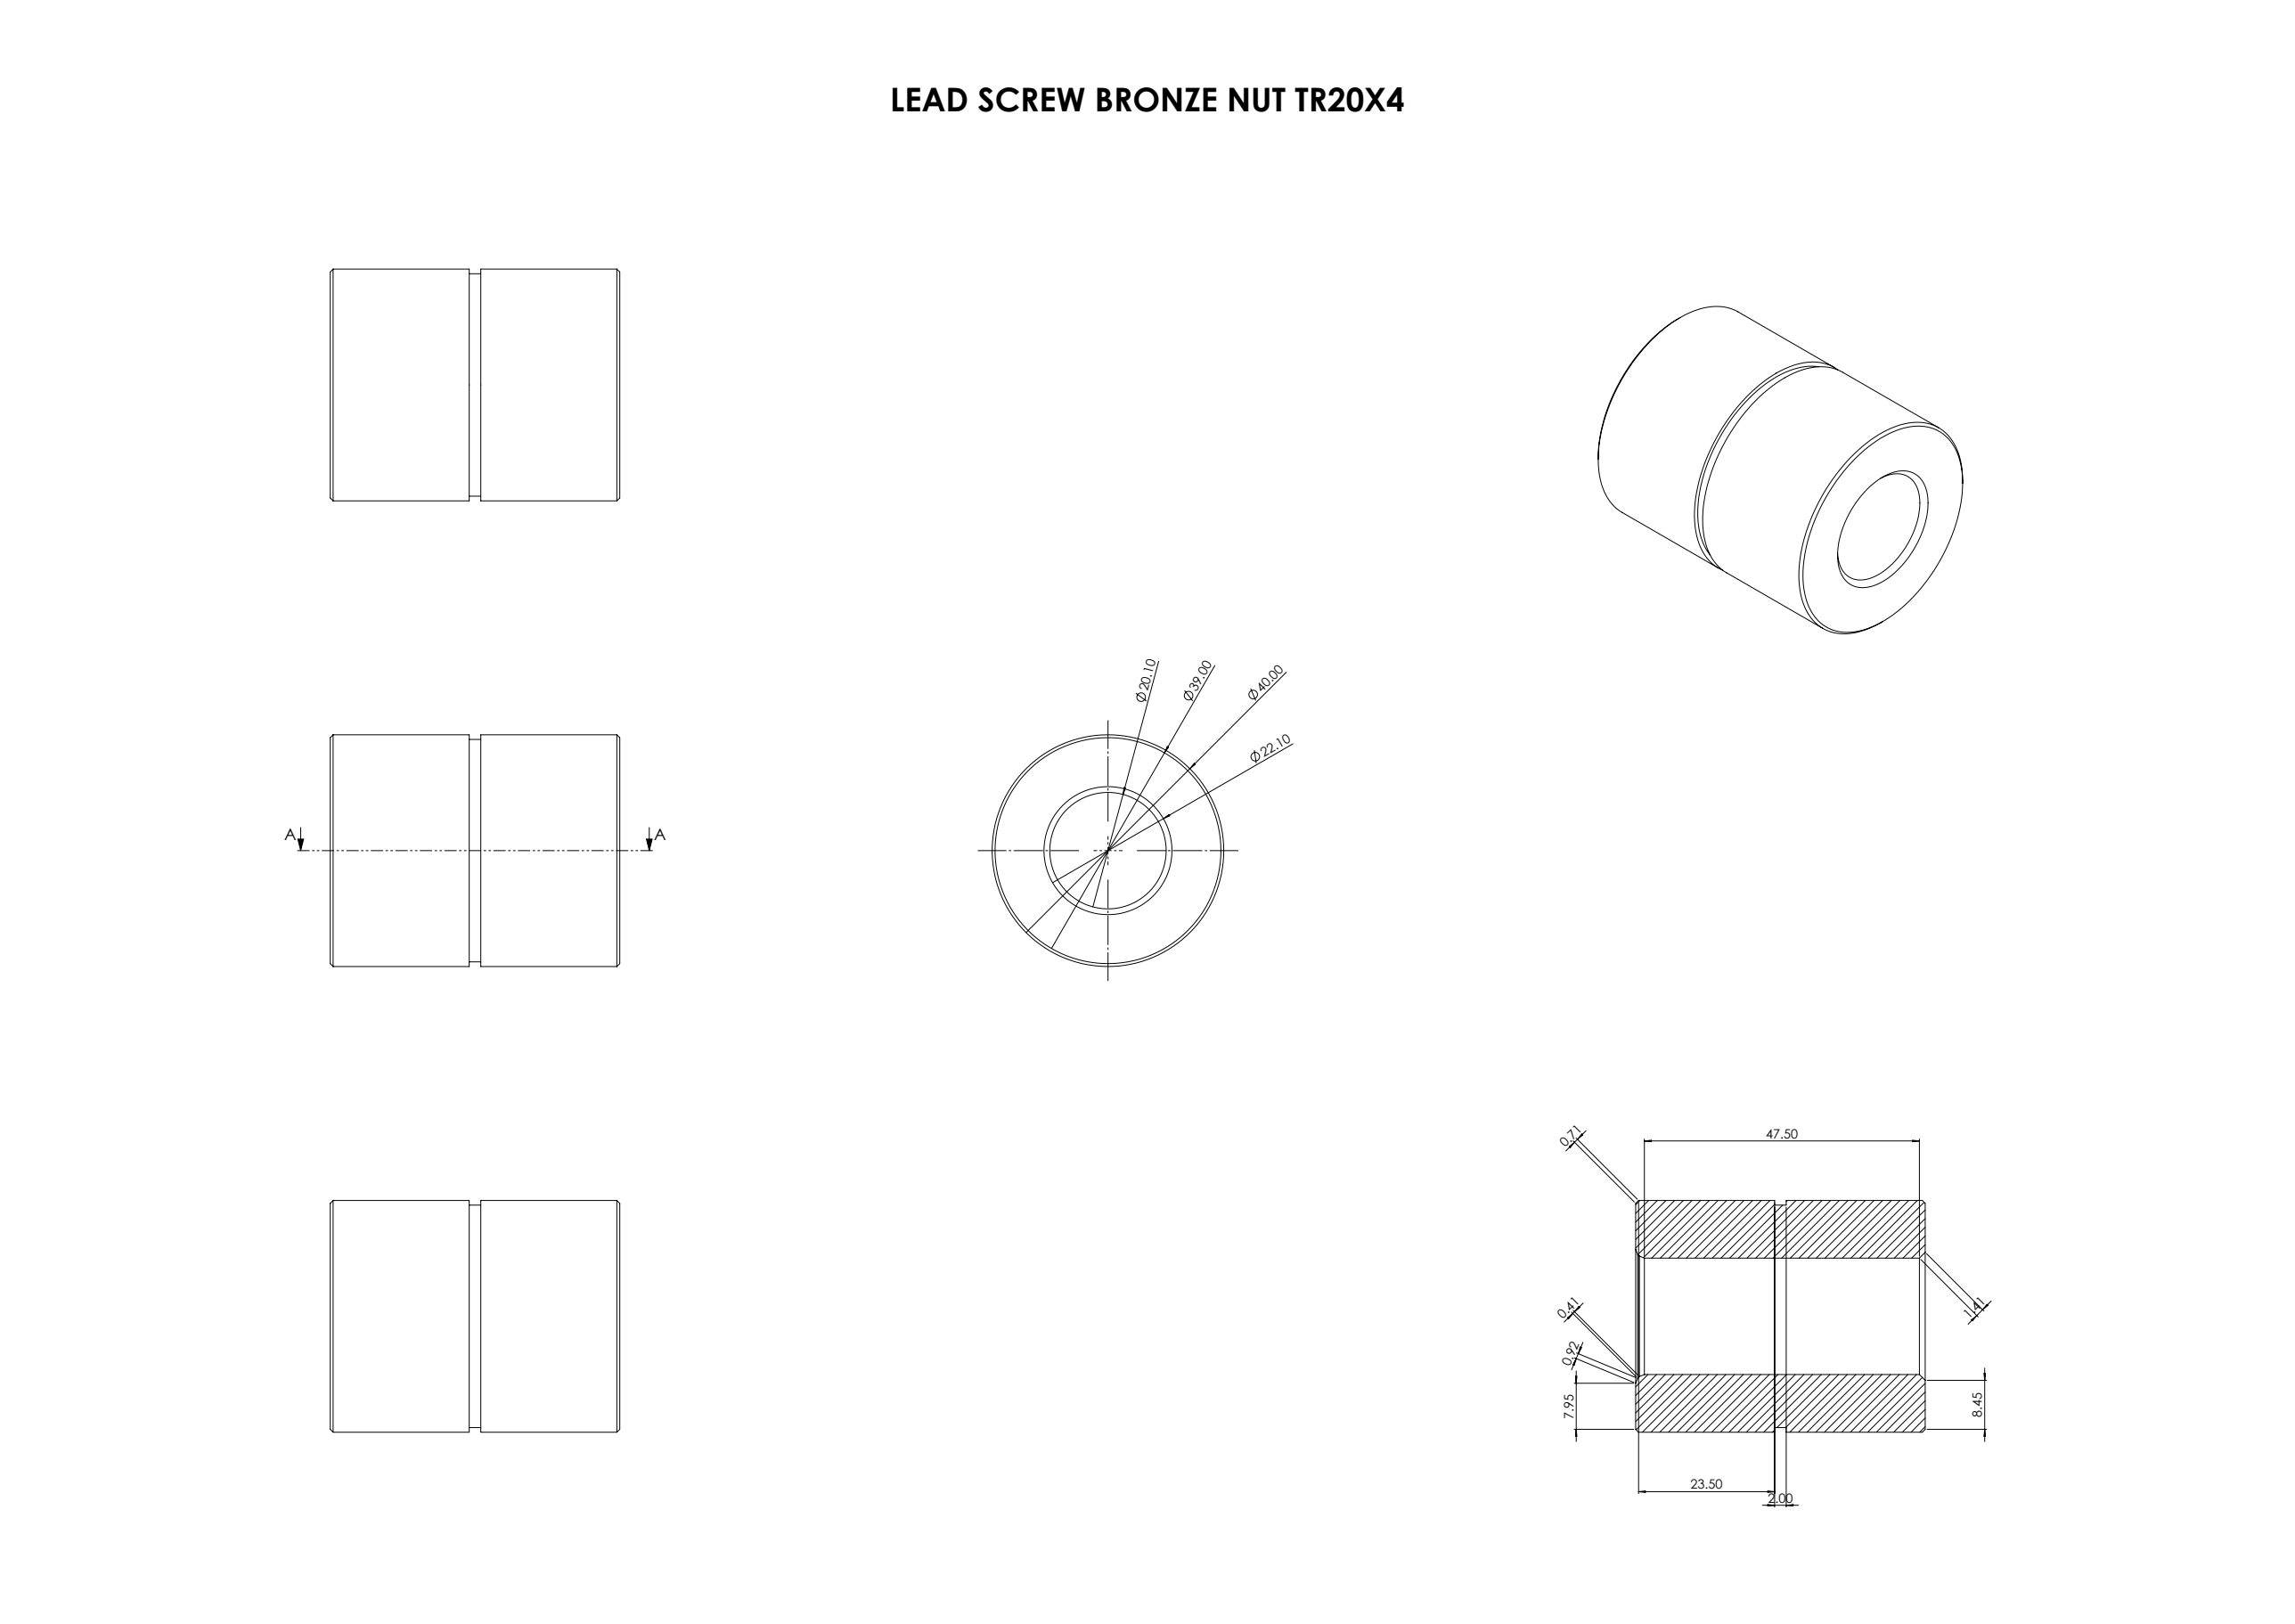
ISO-10303-21;
HEADER;
/* Generated by software containing ST-Developer
 * from STEP Tools, Inc. (www.steptools.com) 
 */

FILE_DESCRIPTION(
/* description */ (''),
/* implementation_level */ '2;1');

FILE_NAME(
/* name */ '06_Lead_Screw_Bronze_Nut_Tr20x4.step',
/* time_stamp */ '2026-10-26T03:50:32-07:00',
/* author */ (''),
/* organization */ (''),
/* preprocessor_version */ 'ST-DEVELOPER v20.2',
/* originating_system */ 'Autodesk Translation Framework v15.15.0.0',
/* authorisation */ '');

FILE_SCHEMA (('AUTOMOTIVE_DESIGN { 1 0 10303 214 3 1 1 }'));
ENDSEC;

DATA;
#10=MECHANICAL_DESIGN_GEOMETRIC_PRESENTATION_REPRESENTATION('',(#1044),#76660);
#1004=SHAPE_REPRESENTATION_RELATIONSHIP('SRR','None',#76741,#1024);
#1024=ADVANCED_BREP_SHAPE_REPRESENTATION('',(#1064),#76645);
#1044=STYLED_ITEM('',(#76913),#1064);
#1064=MANIFOLD_SOLID_BREP('Bronze nut',#26669);
#1251=CYLINDRICAL_SURFACE('',#27734,1.005);
#1252=CYLINDRICAL_SURFACE('',#27739,1.92);
#1253=CYLINDRICAL_SURFACE('',#27743,2.);
#1254=CYLINDRICAL_SURFACE('',#27746,2.);
#1610=FACE_BOUND('',#4683,.T.);
#1611=FACE_BOUND('',#4687,.T.);
#1612=FACE_BOUND('',#4690,.T.);
#1613=FACE_BOUND('',#4696,.T.);
#1925=PLANE('',#27729);
#1926=PLANE('',#27736);
#1927=PLANE('',#27741);
#1928=PLANE('',#27750);
#3071=FACE_OUTER_BOUND('',#4680,.T.);
#3072=FACE_OUTER_BOUND('',#4681,.T.);
#3073=FACE_OUTER_BOUND('',#4682,.T.);
#3074=FACE_OUTER_BOUND('',#4684,.T.);
#3075=FACE_OUTER_BOUND('',#4685,.T.);
#3076=FACE_OUTER_BOUND('',#4686,.T.);
#3077=FACE_OUTER_BOUND('',#4688,.T.);
#3078=FACE_OUTER_BOUND('',#4689,.T.);
#3079=FACE_OUTER_BOUND('',#4691,.T.);
#3080=FACE_OUTER_BOUND('',#4692,.T.);
#3081=FACE_OUTER_BOUND('',#4693,.T.);
#3082=FACE_OUTER_BOUND('',#4694,.T.);
#3083=FACE_OUTER_BOUND('',#4695,.T.);
#3084=FACE_OUTER_BOUND('',#4697,.T.);
#4680=EDGE_LOOP('',(#19859,#19860,#19861,#19862,#19863));
#4681=EDGE_LOOP('',(#19864,#19865,#19866,#19867,#19868,#19869));
#4682=EDGE_LOOP('',(#19870));
#4683=EDGE_LOOP('',(#19871));
#4684=EDGE_LOOP('',(#19872,#19873,#19874,#19875,#19876,#19877));
#4685=EDGE_LOOP('',(#19878,#19879,#19880,#19881,#19882));
#4686=EDGE_LOOP('',(#19883));
#4687=EDGE_LOOP('',(#19884));
#4688=EDGE_LOOP('',(#19885,#19886,#19887,#19888));
#4689=EDGE_LOOP('',(#19889));
#4690=EDGE_LOOP('',(#19890));
#4691=EDGE_LOOP('',(#19891,#19892,#19893,#19894));
#4692=EDGE_LOOP('',(#19895,#19896,#19897,#19898));
#4693=EDGE_LOOP('',(#19899,#19900,#19901,#19902));
#4694=EDGE_LOOP('',(#19903,#19904,#19905,#19906));
#4695=EDGE_LOOP('',(#19907));
#4696=EDGE_LOOP('',(#19908));
#4697=EDGE_LOOP('',(#19909,#19910,#19911,#19912));
#6006=CIRCLE('',#27723,1.155);
#6007=CIRCLE('',#27724,1.06964466094067);
#6008=CIRCLE('',#27725,1.06964466094067);
#6009=CIRCLE('',#27727,1.04035533905933);
#6010=CIRCLE('',#27728,1.04035533905933);
#6011=CIRCLE('',#27730,1.95);
#6012=CIRCLE('',#27732,1.005);
#6013=CIRCLE('',#27733,1.005);
#6014=CIRCLE('',#27735,1.005);
#6015=CIRCLE('',#27737,2.);
#6016=CIRCLE('',#27738,1.92);
#6017=CIRCLE('',#27740,1.92);
#6018=CIRCLE('',#27742,2.);
#6019=CIRCLE('',#27744,2.);
#6020=CIRCLE('',#27747,2.);
#6021=CIRCLE('',#27749,1.95);
#6022=CIRCLE('',#27751,1.105);
#7397=LINE('',#49634,#9553);
#7398=LINE('',#49643,#9554);
#7399=LINE('',#49649,#9555);
#7400=LINE('',#49656,#9556);
#7401=LINE('',#49665,#9557);
#7402=LINE('',#49671,#9558);
#7403=LINE('',#49674,#9559);
#7404=LINE('',#49678,#9560);
#7405=LINE('',#49682,#9561);
#7406=LINE('',#49687,#9562);
#9553=VECTOR('',#31788,1.11232233047034);
#9554=VECTOR('',#31799,1.055);
#9555=VECTOR('',#31806,1.02267766952966);
#9556=VECTOR('',#31815,1.005);
#9557=VECTOR('',#31826,1.92);
#9558=VECTOR('',#31833,2.);
#9559=VECTOR('',#31838,1.975);
#9560=VECTOR('',#31843,2.);
#9561=VECTOR('',#31848,1.975);
#9562=VECTOR('',#31855,1.055);
#11737=VERTEX_POINT('',#49631);
#11738=VERTEX_POINT('',#49633);
#11739=VERTEX_POINT('',#49635);
#11740=VERTEX_POINT('',#49639);
#11741=VERTEX_POINT('',#49640);
#11742=VERTEX_POINT('',#49645);
#11743=VERTEX_POINT('',#49648);
#11744=VERTEX_POINT('',#49650);
#11745=VERTEX_POINT('',#49654);
#11746=VERTEX_POINT('',#49658);
#11747=VERTEX_POINT('',#49660);
#11748=VERTEX_POINT('',#49663);
#11749=VERTEX_POINT('',#49667);
#11750=VERTEX_POINT('',#49670);
#11751=VERTEX_POINT('',#49676);
#11752=VERTEX_POINT('',#49680);
#11753=VERTEX_POINT('',#49684);
#14652=EDGE_CURVE('',#11737,#11737,#6006,.T.);
#14653=EDGE_CURVE('',#11737,#11738,#7397,.T.);
#14654=EDGE_CURVE('',#11738,#11739,#6007,.T.);
#14655=EDGE_CURVE('',#11739,#11738,#6008,.T.);
#14656=EDGE_CURVE('',#11740,#11741,#6009,.T.);
#14657=EDGE_CURVE('',#11741,#11740,#6010,.T.);
#14658=EDGE_CURVE('',#11741,#11739,#7398,.T.);
#14659=EDGE_CURVE('',#11742,#11742,#6011,.T.);
#14660=EDGE_CURVE('',#11740,#11743,#7399,.T.);
#14661=EDGE_CURVE('',#11743,#11744,#6012,.T.);
#14662=EDGE_CURVE('',#11744,#11743,#6013,.T.);
#14663=EDGE_CURVE('',#11745,#11745,#6014,.T.);
#14664=EDGE_CURVE('',#11745,#11744,#7400,.T.);
#14665=EDGE_CURVE('',#11746,#11746,#6015,.T.);
#14666=EDGE_CURVE('',#11747,#11747,#6016,.T.);
#14667=EDGE_CURVE('',#11748,#11748,#6017,.T.);
#14668=EDGE_CURVE('',#11748,#11747,#7401,.T.);
#14669=EDGE_CURVE('',#11749,#11749,#6018,.T.);
#14670=EDGE_CURVE('',#11749,#11750,#7402,.T.);
#14671=EDGE_CURVE('',#11750,#11750,#6019,.T.);
#14672=EDGE_CURVE('',#11750,#11742,#7403,.T.);
#14673=EDGE_CURVE('',#11751,#11751,#6020,.T.);
#14674=EDGE_CURVE('',#11751,#11746,#7404,.T.);
#14675=EDGE_CURVE('',#11752,#11752,#6021,.T.);
#14676=EDGE_CURVE('',#11752,#11751,#7405,.T.);
#14677=EDGE_CURVE('',#11753,#11753,#6022,.T.);
#14678=EDGE_CURVE('',#11753,#11745,#7406,.T.);
#19859=ORIENTED_EDGE('',*,*,#14652,.T.);
#19860=ORIENTED_EDGE('',*,*,#14653,.T.);
#19861=ORIENTED_EDGE('',*,*,#14654,.T.);
#19862=ORIENTED_EDGE('',*,*,#14655,.T.);
#19863=ORIENTED_EDGE('',*,*,#14653,.F.);
#19864=ORIENTED_EDGE('',*,*,#14656,.F.);
#19865=ORIENTED_EDGE('',*,*,#14657,.F.);
#19866=ORIENTED_EDGE('',*,*,#14658,.T.);
#19867=ORIENTED_EDGE('',*,*,#14654,.F.);
#19868=ORIENTED_EDGE('',*,*,#14655,.F.);
#19869=ORIENTED_EDGE('',*,*,#14658,.F.);
#19870=ORIENTED_EDGE('',*,*,#14659,.F.);
#19871=ORIENTED_EDGE('',*,*,#14652,.F.);
#19872=ORIENTED_EDGE('',*,*,#14656,.T.);
#19873=ORIENTED_EDGE('',*,*,#14657,.T.);
#19874=ORIENTED_EDGE('',*,*,#14660,.T.);
#19875=ORIENTED_EDGE('',*,*,#14661,.T.);
#19876=ORIENTED_EDGE('',*,*,#14662,.T.);
#19877=ORIENTED_EDGE('',*,*,#14660,.F.);
#19878=ORIENTED_EDGE('',*,*,#14663,.T.);
#19879=ORIENTED_EDGE('',*,*,#14664,.T.);
#19880=ORIENTED_EDGE('',*,*,#14661,.F.);
#19881=ORIENTED_EDGE('',*,*,#14662,.F.);
#19882=ORIENTED_EDGE('',*,*,#14664,.F.);
#19883=ORIENTED_EDGE('',*,*,#14665,.F.);
#19884=ORIENTED_EDGE('',*,*,#14666,.T.);
#19885=ORIENTED_EDGE('',*,*,#14667,.T.);
#19886=ORIENTED_EDGE('',*,*,#14668,.T.);
#19887=ORIENTED_EDGE('',*,*,#14666,.F.);
#19888=ORIENTED_EDGE('',*,*,#14668,.F.);
#19889=ORIENTED_EDGE('',*,*,#14669,.F.);
#19890=ORIENTED_EDGE('',*,*,#14667,.F.);
#19891=ORIENTED_EDGE('',*,*,#14669,.T.);
#19892=ORIENTED_EDGE('',*,*,#14670,.T.);
#19893=ORIENTED_EDGE('',*,*,#14671,.T.);
#19894=ORIENTED_EDGE('',*,*,#14670,.F.);
#19895=ORIENTED_EDGE('',*,*,#14671,.F.);
#19896=ORIENTED_EDGE('',*,*,#14672,.T.);
#19897=ORIENTED_EDGE('',*,*,#14659,.T.);
#19898=ORIENTED_EDGE('',*,*,#14672,.F.);
#19899=ORIENTED_EDGE('',*,*,#14673,.F.);
#19900=ORIENTED_EDGE('',*,*,#14674,.T.);
#19901=ORIENTED_EDGE('',*,*,#14665,.T.);
#19902=ORIENTED_EDGE('',*,*,#14674,.F.);
#19903=ORIENTED_EDGE('',*,*,#14675,.F.);
#19904=ORIENTED_EDGE('',*,*,#14676,.T.);
#19905=ORIENTED_EDGE('',*,*,#14673,.T.);
#19906=ORIENTED_EDGE('',*,*,#14676,.F.);
#19907=ORIENTED_EDGE('',*,*,#14675,.T.);
#19908=ORIENTED_EDGE('',*,*,#14677,.F.);
#19909=ORIENTED_EDGE('',*,*,#14677,.T.);
#19910=ORIENTED_EDGE('',*,*,#14678,.T.);
#19911=ORIENTED_EDGE('',*,*,#14663,.F.);
#19912=ORIENTED_EDGE('',*,*,#14678,.F.);
#25027=CONICAL_SURFACE('',#27722,1.11232233047034,1.17809724509617);
#25028=CONICAL_SURFACE('',#27726,1.055,0.78539816339745);
#25029=CONICAL_SURFACE('',#27731,1.02267766952966,0.39269908169873);
#25030=CONICAL_SURFACE('',#27745,1.975,0.785398163397442);
#25031=CONICAL_SURFACE('',#27748,1.975,0.785398163397442);
#25032=CONICAL_SURFACE('',#27752,1.055,0.78539816339745);
#25659=ADVANCED_FACE('',(#3071),#25027,.F.);
#25660=ADVANCED_FACE('',(#3072),#25028,.F.);
#25661=ADVANCED_FACE('',(#3073,#1610),#1925,.T.);
#25662=ADVANCED_FACE('',(#3074),#25029,.F.);
#25663=ADVANCED_FACE('',(#3075),#1251,.F.);
#25664=ADVANCED_FACE('',(#3076,#1611),#1926,.F.);
#25665=ADVANCED_FACE('',(#3077),#1252,.T.);
#25666=ADVANCED_FACE('',(#3078,#1612),#1927,.F.);
#25667=ADVANCED_FACE('',(#3079),#1253,.T.);
#25668=ADVANCED_FACE('',(#3080),#25030,.T.);
#25669=ADVANCED_FACE('',(#3081),#1254,.T.);
#25670=ADVANCED_FACE('',(#3082),#25031,.T.);
#25671=ADVANCED_FACE('',(#3083,#1613),#1928,.T.);
#25672=ADVANCED_FACE('',(#3084),#25032,.F.);
#26669=CLOSED_SHELL('',(#25659,#25660,#25661,#25662,#25663,#25664,#25665,
#25666,#25667,#25668,#25669,#25670,#25671,#25672));
#27721=AXIS2_PLACEMENT_3D('',#49629,#31782,#31783);
#27722=AXIS2_PLACEMENT_3D('',#49630,#31784,#31785);
#27723=AXIS2_PLACEMENT_3D('',#49632,#31786,#31787);
#27724=AXIS2_PLACEMENT_3D('',#49636,#31789,#31790);
#27725=AXIS2_PLACEMENT_3D('',#49637,#31791,#31792);
#27726=AXIS2_PLACEMENT_3D('',#49638,#31793,#31794);
#27727=AXIS2_PLACEMENT_3D('',#49641,#31795,#31796);
#27728=AXIS2_PLACEMENT_3D('',#49642,#31797,#31798);
#27729=AXIS2_PLACEMENT_3D('',#49644,#31800,#31801);
#27730=AXIS2_PLACEMENT_3D('',#49646,#31802,#31803);
#27731=AXIS2_PLACEMENT_3D('',#49647,#31804,#31805);
#27732=AXIS2_PLACEMENT_3D('',#49651,#31807,#31808);
#27733=AXIS2_PLACEMENT_3D('',#49652,#31809,#31810);
#27734=AXIS2_PLACEMENT_3D('',#49653,#31811,#31812);
#27735=AXIS2_PLACEMENT_3D('',#49655,#31813,#31814);
#27736=AXIS2_PLACEMENT_3D('',#49657,#31816,#31817);
#27737=AXIS2_PLACEMENT_3D('',#49659,#31818,#31819);
#27738=AXIS2_PLACEMENT_3D('',#49661,#31820,#31821);
#27739=AXIS2_PLACEMENT_3D('',#49662,#31822,#31823);
#27740=AXIS2_PLACEMENT_3D('',#49664,#31824,#31825);
#27741=AXIS2_PLACEMENT_3D('',#49666,#31827,#31828);
#27742=AXIS2_PLACEMENT_3D('',#49668,#31829,#31830);
#27743=AXIS2_PLACEMENT_3D('',#49669,#31831,#31832);
#27744=AXIS2_PLACEMENT_3D('',#49672,#31834,#31835);
#27745=AXIS2_PLACEMENT_3D('',#49673,#31836,#31837);
#27746=AXIS2_PLACEMENT_3D('',#49675,#31839,#31840);
#27747=AXIS2_PLACEMENT_3D('',#49677,#31841,#31842);
#27748=AXIS2_PLACEMENT_3D('',#49679,#31844,#31845);
#27749=AXIS2_PLACEMENT_3D('',#49681,#31846,#31847);
#27750=AXIS2_PLACEMENT_3D('',#49683,#31849,#31850);
#27751=AXIS2_PLACEMENT_3D('',#49685,#31851,#31852);
#27752=AXIS2_PLACEMENT_3D('',#49686,#31853,#31854);
#31782=DIRECTION('axis',(0.,0.,1.));
#31783=DIRECTION('refdir',(1.,0.,0.));
#31784=DIRECTION('center_axis',(-1.,0.,0.));
#31785=DIRECTION('ref_axis',(0.,-1.,0.));
#31786=DIRECTION('center_axis',(-1.,0.,0.));
#31787=DIRECTION('ref_axis',(0.,-1.,0.));
#31788=DIRECTION('',(0.382683432365091,-0.923879532511286,1.1314261122877E-16));
#31789=DIRECTION('center_axis',(1.,0.,-1.66069808438821E-15));
#31790=DIRECTION('ref_axis',(0.,-1.,0.));
#31791=DIRECTION('center_axis',(1.,0.,-1.66069808438821E-15));
#31792=DIRECTION('ref_axis',(0.,-1.,0.));
#31793=DIRECTION('center_axis',(-1.,0.,0.));
#31794=DIRECTION('ref_axis',(0.,1.,0.));
#31795=DIRECTION('center_axis',(-1.,0.,0.));
#31796=DIRECTION('ref_axis',(0.,-1.,0.));
#31797=DIRECTION('center_axis',(-1.,0.,0.));
#31798=DIRECTION('ref_axis',(0.,-1.,0.));
#31799=DIRECTION('',(-0.707106781186547,-0.707106781186548,-8.65956056235494E-17));
#31800=DIRECTION('center_axis',(-1.,0.,0.));
#31801=DIRECTION('ref_axis',(0.,0.,1.));
#31802=DIRECTION('center_axis',(1.,0.,0.));
#31803=DIRECTION('ref_axis',(0.,0.,-1.));
#31804=DIRECTION('center_axis',(-1.,0.,0.));
#31805=DIRECTION('ref_axis',(0.,-1.,0.));
#31806=DIRECTION('',(0.923879532511285,-0.382683432365095,4.68652040532636E-17));
#31807=DIRECTION('center_axis',(1.,0.,0.));
#31808=DIRECTION('ref_axis',(0.,-1.,0.));
#31809=DIRECTION('center_axis',(1.,0.,0.));
#31810=DIRECTION('ref_axis',(0.,-1.,0.));
#31811=DIRECTION('center_axis',(1.,0.,0.));
#31812=DIRECTION('ref_axis',(0.,1.,0.));
#31813=DIRECTION('center_axis',(1.,0.,0.));
#31814=DIRECTION('ref_axis',(0.,0.,-1.));
#31815=DIRECTION('',(-1.,0.,0.));
#31816=DIRECTION('center_axis',(1.,0.,0.));
#31817=DIRECTION('ref_axis',(0.,0.,-1.));
#31818=DIRECTION('center_axis',(1.,0.,0.));
#31819=DIRECTION('ref_axis',(0.,1.,0.));
#31820=DIRECTION('center_axis',(1.,0.,0.));
#31821=DIRECTION('ref_axis',(0.,0.,-1.));
#31822=DIRECTION('center_axis',(1.,0.,0.));
#31823=DIRECTION('ref_axis',(0.,1.,0.));
#31824=DIRECTION('center_axis',(1.,0.,0.));
#31825=DIRECTION('ref_axis',(0.,0.,-1.));
#31826=DIRECTION('',(1.,0.,0.));
#31827=DIRECTION('center_axis',(-1.,0.,0.));
#31828=DIRECTION('ref_axis',(0.,0.,1.));
#31829=DIRECTION('center_axis',(-1.,0.,0.));
#31830=DIRECTION('ref_axis',(0.,1.,0.));
#31831=DIRECTION('center_axis',(1.,0.,0.));
#31832=DIRECTION('ref_axis',(0.,1.,0.));
#31833=DIRECTION('',(-1.,0.,0.));
#31834=DIRECTION('center_axis',(1.,0.,0.));
#31835=DIRECTION('ref_axis',(0.,0.,-1.));
#31836=DIRECTION('center_axis',(1.,0.,0.));
#31837=DIRECTION('ref_axis',(0.,1.,0.));
#31838=DIRECTION('',(-0.707106781186552,0.707106781186543,8.65956056235488E-17));
#31839=DIRECTION('center_axis',(1.,0.,0.));
#31840=DIRECTION('ref_axis',(0.,1.,0.));
#31841=DIRECTION('center_axis',(1.,0.,0.));
#31842=DIRECTION('ref_axis',(0.,0.,-1.));
#31843=DIRECTION('',(-1.,0.,0.));
#31844=DIRECTION('center_axis',(-1.,0.,0.));
#31845=DIRECTION('ref_axis',(0.,1.,0.));
#31846=DIRECTION('center_axis',(1.,0.,0.));
#31847=DIRECTION('ref_axis',(0.,0.,-1.));
#31848=DIRECTION('',(-0.707106781186552,-0.707106781186543,-8.65956056235488E-17));
#31849=DIRECTION('center_axis',(1.,0.,0.));
#31850=DIRECTION('ref_axis',(0.,0.,-1.));
#31851=DIRECTION('center_axis',(1.,0.,0.));
#31852=DIRECTION('ref_axis',(0.,0.,-1.));
#31853=DIRECTION('center_axis',(1.,0.,0.));
#31854=DIRECTION('ref_axis',(0.,1.,0.));
#31855=DIRECTION('',(-0.707106781186547,0.707106781186548,8.65956056235494E-17));
#49629=CARTESIAN_POINT('',(0.,0.,0.));
#49630=CARTESIAN_POINT('Origin',(10.0176776695297,0.,26.5));
#49631=CARTESIAN_POINT('',(10.,1.155,26.5));
#49632=CARTESIAN_POINT('Origin',(10.,0.,26.5));
#49633=CARTESIAN_POINT('',(10.0353553390593,1.06964466094067,26.5));
#49634=CARTESIAN_POINT('',(10.0176776695297,1.11232233047034,26.5));
#49635=CARTESIAN_POINT('',(10.0353553390593,-1.06964466094068,26.5));
#49636=CARTESIAN_POINT('Origin',(10.0353553390593,0.,26.5));
#49637=CARTESIAN_POINT('Origin',(10.0353553390593,0.,26.5));
#49638=CARTESIAN_POINT('Origin',(10.05,0.,26.5));
#49639=CARTESIAN_POINT('',(10.0646446609407,1.04035533905933,26.5));
#49640=CARTESIAN_POINT('',(10.0646446609407,-1.04035533905933,26.5));
#49641=CARTESIAN_POINT('Origin',(10.0646446609407,0.,26.5));
#49642=CARTESIAN_POINT('Origin',(10.0646446609407,0.,26.5));
#49643=CARTESIAN_POINT('',(10.05,-1.055,26.5));
#49644=CARTESIAN_POINT('Origin',(10.,1.95,26.5));
#49645=CARTESIAN_POINT('',(10.,-1.95,26.5));
#49646=CARTESIAN_POINT('Origin',(10.,0.,26.5));
#49647=CARTESIAN_POINT('Origin',(10.1073223304703,0.,26.5));
#49648=CARTESIAN_POINT('',(10.15,1.005,26.5));
#49649=CARTESIAN_POINT('',(10.1073223304703,1.02267766952966,26.5));
#49650=CARTESIAN_POINT('',(10.15,-1.005,26.5));
#49651=CARTESIAN_POINT('Origin',(10.15,0.,26.5));
#49652=CARTESIAN_POINT('Origin',(10.15,0.,26.5));
#49653=CARTESIAN_POINT('Origin',(12.5,0.,26.5));
#49654=CARTESIAN_POINT('',(14.9,-1.005,26.5));
#49655=CARTESIAN_POINT('Origin',(14.9,0.,26.5));
#49656=CARTESIAN_POINT('',(12.5,-1.005,26.5));
#49657=CARTESIAN_POINT('Origin',(12.6,1.92,26.5));
#49658=CARTESIAN_POINT('',(12.6,-2.,26.5));
#49659=CARTESIAN_POINT('Origin',(12.6,0.,26.5));
#49660=CARTESIAN_POINT('',(12.6,-1.92,26.5));
#49661=CARTESIAN_POINT('Origin',(12.6,0.,26.5));
#49662=CARTESIAN_POINT('Origin',(12.5,0.,26.5));
#49663=CARTESIAN_POINT('',(12.4,-1.92,26.5));
#49664=CARTESIAN_POINT('Origin',(12.4,0.,26.5));
#49665=CARTESIAN_POINT('',(12.5,-1.92,26.5));
#49666=CARTESIAN_POINT('Origin',(12.4,2.01,26.5));
#49667=CARTESIAN_POINT('',(12.4,-2.,26.5));
#49668=CARTESIAN_POINT('Origin',(12.4,0.,26.5));
#49669=CARTESIAN_POINT('Origin',(12.5,0.,26.5));
#49670=CARTESIAN_POINT('',(10.05,-2.,26.5));
#49671=CARTESIAN_POINT('',(12.5,-2.,26.5));
#49672=CARTESIAN_POINT('Origin',(10.05,0.,26.5));
#49673=CARTESIAN_POINT('Origin',(10.025,0.,26.5));
#49674=CARTESIAN_POINT('',(10.025,-1.975,26.5));
#49675=CARTESIAN_POINT('Origin',(12.5,0.,26.5));
#49676=CARTESIAN_POINT('',(14.95,-2.,26.5));
#49677=CARTESIAN_POINT('Origin',(14.95,0.,26.5));
#49678=CARTESIAN_POINT('',(12.5,-2.,26.5));
#49679=CARTESIAN_POINT('Origin',(14.975,0.,26.5));
#49680=CARTESIAN_POINT('',(15.,-1.95,26.5));
#49681=CARTESIAN_POINT('Origin',(15.,0.,26.5));
#49682=CARTESIAN_POINT('',(14.975,-1.975,26.5));
#49683=CARTESIAN_POINT('Origin',(15.,1.105,26.5));
#49684=CARTESIAN_POINT('',(15.,-1.105,26.5));
#49685=CARTESIAN_POINT('Origin',(15.,0.,26.5));
#49686=CARTESIAN_POINT('Origin',(14.95,0.,26.5));
#49687=CARTESIAN_POINT('',(14.95,-1.055,26.5));
#76623=UNCERTAINTY_MEASURE_WITH_UNIT(LENGTH_MEASURE(0.001),#76661,
'DISTANCE_ACCURACY_VALUE',
'Maximum model space distance between geometric entities at asserted c
onnectivities');
#76638=UNCERTAINTY_MEASURE_WITH_UNIT(LENGTH_MEASURE(0.001),#76661,
'DISTANCE_ACCURACY_VALUE',
'Maximum model space distance between geometric entities at asserted c
onnectivities');
#76645=(
GEOMETRIC_REPRESENTATION_CONTEXT(3)
GLOBAL_UNCERTAINTY_ASSIGNED_CONTEXT((#76623))
GLOBAL_UNIT_ASSIGNED_CONTEXT((#76661,#76663,#76664))
REPRESENTATION_CONTEXT('','3D')
);
#76660=(
GEOMETRIC_REPRESENTATION_CONTEXT(3)
GLOBAL_UNCERTAINTY_ASSIGNED_CONTEXT((#76638))
GLOBAL_UNIT_ASSIGNED_CONTEXT((#76661,#76663,#76664))
REPRESENTATION_CONTEXT('','3D')
);
#76661=(
LENGTH_UNIT()
NAMED_UNIT(*)
SI_UNIT(.CENTI.,.METRE.)
);
#76663=(
NAMED_UNIT(*)
PLANE_ANGLE_UNIT()
SI_UNIT($,.RADIAN.)
);
#76664=(
NAMED_UNIT(*)
SI_UNIT($,.STERADIAN.)
SOLID_ANGLE_UNIT()
);
#76671=SHAPE_DEFINITION_REPRESENTATION(#76692,#76741);
#76692=PRODUCT_DEFINITION_SHAPE('',$,#76763);
#76741=SHAPE_REPRESENTATION('',(#27721),#76645);
#76756=PRODUCT_DEFINITION_CONTEXT('part definition',#76821,'design');
#76763=PRODUCT_DEFINITION('2026-10-26-11-12-47-434',
'06_Lead_Screw_Bronze_Nut_Tr20x4',#76784,#76756);
#76784=PRODUCT_DEFINITION_FORMATION('',$,#76829);
#76821=APPLICATION_CONTEXT(
'Core Data for Automotive Mechanical Design Process');
#76822=PRODUCT_CONTEXT('part definition',#76821,'mechanical');
#76829=PRODUCT('2026-10-26-11-12-47-434',
'06_Lead_Screw_Bronze_Nut_Tr20x4',$,(#76822));
#76907=COLOUR_RGB('Black',0.12,0.14,0.17);
#76908=FILL_AREA_STYLE_COLOUR('',#76907);
#76909=FILL_AREA_STYLE('',(#76908));
#76910=SURFACE_STYLE_FILL_AREA(#76909);
#76911=SURFACE_SIDE_STYLE('',(#76910));
#76912=SURFACE_STYLE_USAGE(.BOTH.,#76911);
#76913=PRESENTATION_STYLE_ASSIGNMENT((#76912));
ENDSEC;
END-ISO-10303-21;
